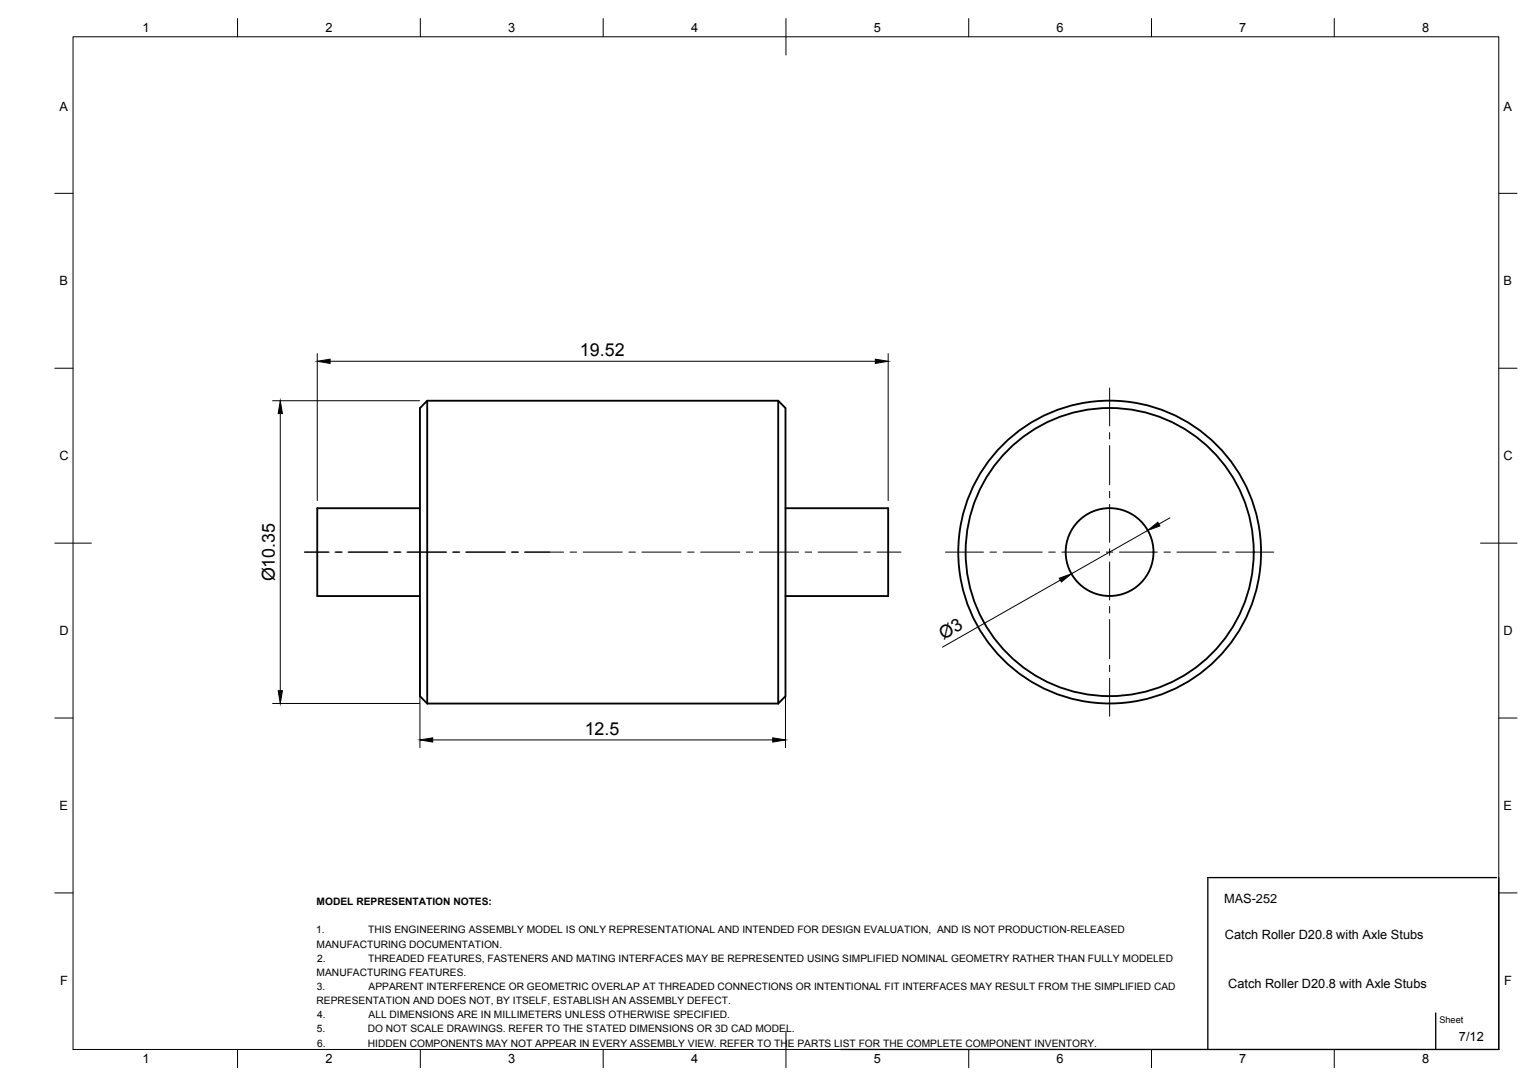
ISO-10303-21;
HEADER;
FILE_DESCRIPTION((''),'2;1');
FILE_NAME('Catch Roller D20.8 with Axle Stubs.step','2026-10-06T07:01:46+05:00',(''),(''),'','','');
FILE_SCHEMA (('AUTOMOTIVE_DESIGN { 1 0 10303 214 3 1 1 }'));
ENDSEC;
DATA;
#10=MECHANICAL_DESIGN_GEOMETRIC_PRESENTATION_REPRESENTATION('',(#142),#11396);
#97=CONICAL_SURFACE('',#6232,5.05,0.785398163397455) ;
#98=CONICAL_SURFACE('',#6236,5.05,0.785398163397455) ;
#112=SHAPE_REPRESENTATION_RELATIONSHIP('SRR','None',#11459,#127) ;
#127=ADVANCED_BREP_SHAPE_REPRESENTATION('',(#157),#11385) ;
#142=STYLED_ITEM('',(#11543),#157) ;
#157=MANIFOLD_SOLID_BREP('Catch Roller D20.8 with Axle Stubs',#5573) ;
#363=FACE_BOUND('',#1122,.T.) ;
#364=FACE_BOUND('',#1127,.T.) ;
#462=PLANE('',#6226) ;
#463=PLANE('',#6230) ;
#464=PLANE('',#6238) ;
#465=PLANE('',#6242) ;
#757=FACE_OUTER_BOUND('',#1119,.T.) ;
#758=FACE_OUTER_BOUND('',#1120,.T.) ;
#759=FACE_OUTER_BOUND('',#1121,.T.) ;
#760=FACE_OUTER_BOUND('',#1123,.T.) ;
#761=FACE_OUTER_BOUND('',#1124,.T.) ;
#762=FACE_OUTER_BOUND('',#1125,.T.) ;
#763=FACE_OUTER_BOUND('',#1126,.T.) ;
#764=FACE_OUTER_BOUND('',#1128,.T.) ;
#765=FACE_OUTER_BOUND('',#1129,.T.) ;
#1119=EDGE_LOOP('',(#4726)) ;
#1120=EDGE_LOOP('',(#4727,#4728,#4729,#4730)) ;
#1121=EDGE_LOOP('',(#4731)) ;
#1122=EDGE_LOOP('',(#4732)) ;
#1123=EDGE_LOOP('',(#4733,#4734,#4735,#4736)) ;
#1124=EDGE_LOOP('',(#4737,#4738,#4739,#4740)) ;
#1125=EDGE_LOOP('',(#4741,#4742,#4743,#4744)) ;
#1126=EDGE_LOOP('',(#4745)) ;
#1127=EDGE_LOOP('',(#4746)) ;
#1128=EDGE_LOOP('',(#4747,#4748,#4749,#4750)) ;
#1129=EDGE_LOOP('',(#4751)) ;
#1498=LINE('',#10819,#1881) ;
#1499=LINE('',#10826,#1882) ;
#1500=LINE('',#10830,#1883) ;
#1501=LINE('',#10834,#1884) ;
#1502=LINE('',#10841,#1885) ;
#1881=VECTOR('',#7652,1.5) ;
#1882=VECTOR('',#7661,5.05) ;
#1883=VECTOR('',#7666,5.175) ;
#1884=VECTOR('',#7671,5.05) ;
#1885=VECTOR('',#7680,1.5) ;
#2198=CIRCLE('',#6227,1.5) ;
#2199=CIRCLE('',#6229,1.5) ;
#2200=CIRCLE('',#6231,4.925) ;
#2201=CIRCLE('',#6233,5.175) ;
#2202=CIRCLE('',#6235,5.175) ;
#2203=CIRCLE('',#6237,4.925) ;
#2204=CIRCLE('',#6239,1.5) ;
#2205=CIRCLE('',#6241,1.5) ;
#2627=VERTEX_POINT('',#10814) ;
#2628=VERTEX_POINT('',#10817) ;
#2629=VERTEX_POINT('',#10821) ;
#2630=VERTEX_POINT('',#10824) ;
#2631=VERTEX_POINT('',#10828) ;
#2632=VERTEX_POINT('',#10832) ;
#2633=VERTEX_POINT('',#10836) ;
#2634=VERTEX_POINT('',#10839) ;
#3345=EDGE_CURVE('',#2627,#2627,#2198,.T.) ;
#3346=EDGE_CURVE('',#2628,#2628,#2199,.T.) ;
#3347=EDGE_CURVE('',#2628,#2627,#1498,.T.) ;
#3348=EDGE_CURVE('',#2629,#2629,#2200,.T.) ;
#3349=EDGE_CURVE('',#2630,#2630,#2201,.T.) ;
#3350=EDGE_CURVE('',#2630,#2629,#1499,.T.) ;
#3351=EDGE_CURVE('',#2631,#2631,#2202,.T.) ;
#3352=EDGE_CURVE('',#2631,#2630,#1500,.T.) ;
#3353=EDGE_CURVE('',#2632,#2632,#2203,.T.) ;
#3354=EDGE_CURVE('',#2632,#2631,#1501,.T.) ;
#3355=EDGE_CURVE('',#2633,#2633,#2204,.T.) ;
#3356=EDGE_CURVE('',#2634,#2634,#2205,.T.) ;
#3357=EDGE_CURVE('',#2634,#2633,#1502,.T.) ;
#4726=ORIENTED_EDGE('',*,*,#3345,.F.) ;
#4727=ORIENTED_EDGE('',*,*,#3346,.F.) ;
#4728=ORIENTED_EDGE('',*,*,#3347,.T.) ;
#4729=ORIENTED_EDGE('',*,*,#3345,.T.) ;
#4730=ORIENTED_EDGE('',*,*,#3347,.F.) ;
#4731=ORIENTED_EDGE('',*,*,#3348,.F.) ;
#4732=ORIENTED_EDGE('',*,*,#3346,.T.) ;
#4733=ORIENTED_EDGE('',*,*,#3349,.F.) ;
#4734=ORIENTED_EDGE('',*,*,#3350,.T.) ;
#4735=ORIENTED_EDGE('',*,*,#3348,.T.) ;
#4736=ORIENTED_EDGE('',*,*,#3350,.F.) ;
#4737=ORIENTED_EDGE('',*,*,#3351,.F.) ;
#4738=ORIENTED_EDGE('',*,*,#3352,.T.) ;
#4739=ORIENTED_EDGE('',*,*,#3349,.T.) ;
#4740=ORIENTED_EDGE('',*,*,#3352,.F.) ;
#4741=ORIENTED_EDGE('',*,*,#3353,.F.) ;
#4742=ORIENTED_EDGE('',*,*,#3354,.T.) ;
#4743=ORIENTED_EDGE('',*,*,#3351,.T.) ;
#4744=ORIENTED_EDGE('',*,*,#3354,.F.) ;
#4745=ORIENTED_EDGE('',*,*,#3353,.T.) ;
#4746=ORIENTED_EDGE('',*,*,#3355,.F.) ;
#4747=ORIENTED_EDGE('',*,*,#3356,.F.) ;
#4748=ORIENTED_EDGE('',*,*,#3357,.T.) ;
#4749=ORIENTED_EDGE('',*,*,#3355,.T.) ;
#4750=ORIENTED_EDGE('',*,*,#3357,.F.) ;
#4751=ORIENTED_EDGE('',*,*,#3356,.T.) ;
#5205=CYLINDRICAL_SURFACE('',#6228,1.5) ;
#5206=CYLINDRICAL_SURFACE('',#6234,5.175) ;
#5207=CYLINDRICAL_SURFACE('',#6240,1.5) ;
#5482=ADVANCED_FACE('',(#757),#462,.T.) ;
#5483=ADVANCED_FACE('',(#758),#5205,.T.) ;
#5484=ADVANCED_FACE('',(#759,#363),#463,.T.) ;
#5485=ADVANCED_FACE('',(#760),#97,.T.) ;
#5486=ADVANCED_FACE('',(#761),#5206,.T.) ;
#5487=ADVANCED_FACE('',(#762),#98,.T.) ;
#5488=ADVANCED_FACE('',(#763,#364),#464,.T.) ;
#5489=ADVANCED_FACE('',(#764),#5207,.T.) ;
#5490=ADVANCED_FACE('',(#765),#465,.T.) ;
#5573=CLOSED_SHELL('',(#5482,#5483,#5484,#5485,#5486,#5487,#5488,#5489,
#5490)) ;
#6225=AXIS2_PLACEMENT_3D('',#10812,#7642,#7643) ;
#6226=AXIS2_PLACEMENT_3D('',#10813,#7644,#7645) ;
#6227=AXIS2_PLACEMENT_3D('',#10815,#7646,#7647) ;
#6228=AXIS2_PLACEMENT_3D('',#10816,#7648,#7649) ;
#6229=AXIS2_PLACEMENT_3D('',#10818,#7650,#7651) ;
#6230=AXIS2_PLACEMENT_3D('',#10820,#7653,#7654) ;
#6231=AXIS2_PLACEMENT_3D('',#10822,#7655,#7656) ;
#6232=AXIS2_PLACEMENT_3D('',#10823,#7657,#7658) ;
#6233=AXIS2_PLACEMENT_3D('',#10825,#7659,#7660) ;
#6234=AXIS2_PLACEMENT_3D('',#10827,#7662,#7663) ;
#6235=AXIS2_PLACEMENT_3D('',#10829,#7664,#7665) ;
#6236=AXIS2_PLACEMENT_3D('',#10831,#7667,#7668) ;
#6237=AXIS2_PLACEMENT_3D('',#10833,#7669,#7670) ;
#6238=AXIS2_PLACEMENT_3D('',#10835,#7672,#7673) ;
#6239=AXIS2_PLACEMENT_3D('',#10837,#7674,#7675) ;
#6240=AXIS2_PLACEMENT_3D('',#10838,#7676,#7677) ;
#6241=AXIS2_PLACEMENT_3D('',#10840,#7678,#7679) ;
#6242=AXIS2_PLACEMENT_3D('',#10842,#7681,#7682) ;
#7642=DIRECTION('axis',(0.,0.,1.)) ;
#7643=DIRECTION('refdir',(1.,0.,0.)) ;
#7644=DIRECTION('center_axis',(-1.,0.,0.)) ;
#7645=DIRECTION('ref_axis',(0.,0.,1.)) ;
#7646=DIRECTION('center_axis',(1.,0.,0.)) ;
#7647=DIRECTION('ref_axis',(0.,0.,-1.)) ;
#7648=DIRECTION('center_axis',(1.,0.,0.)) ;
#7649=DIRECTION('ref_axis',(0.,1.,0.)) ;
#7650=DIRECTION('center_axis',(1.,0.,0.)) ;
#7651=DIRECTION('ref_axis',(0.,0.,-1.)) ;
#7652=DIRECTION('',(-1.,0.,0.)) ;
#7653=DIRECTION('center_axis',(-1.,0.,0.)) ;
#7654=DIRECTION('ref_axis',(0.,0.,1.)) ;
#7655=DIRECTION('center_axis',(1.,0.,0.)) ;
#7656=DIRECTION('ref_axis',(0.,0.,-1.)) ;
#7657=DIRECTION('center_axis',(1.,0.,0.)) ;
#7658=DIRECTION('ref_axis',(0.,1.,0.)) ;
#7659=DIRECTION('center_axis',(1.,0.,0.)) ;
#7660=DIRECTION('ref_axis',(0.,0.,-1.)) ;
#7661=DIRECTION('',(-0.707106781186543,0.707106781186552,8.65956056235499E-17)) ;
#7662=DIRECTION('center_axis',(1.,0.,0.)) ;
#7663=DIRECTION('ref_axis',(0.,1.,0.)) ;
#7664=DIRECTION('center_axis',(1.,0.,0.)) ;
#7665=DIRECTION('ref_axis',(0.,0.,-1.)) ;
#7666=DIRECTION('',(-1.,0.,0.)) ;
#7667=DIRECTION('center_axis',(-1.,0.,0.)) ;
#7668=DIRECTION('ref_axis',(0.,1.,0.)) ;
#7669=DIRECTION('center_axis',(1.,0.,0.)) ;
#7670=DIRECTION('ref_axis',(0.,0.,-1.)) ;
#7671=DIRECTION('',(-0.707106781186543,-0.707106781186552,-8.65956056235499E-17)) ;
#7672=DIRECTION('center_axis',(1.,0.,0.)) ;
#7673=DIRECTION('ref_axis',(0.,0.,-1.)) ;
#7674=DIRECTION('center_axis',(1.,0.,0.)) ;
#7675=DIRECTION('ref_axis',(0.,0.,-1.)) ;
#7676=DIRECTION('center_axis',(1.,0.,0.)) ;
#7677=DIRECTION('ref_axis',(0.,1.,0.)) ;
#7678=DIRECTION('center_axis',(1.,0.,0.)) ;
#7679=DIRECTION('ref_axis',(0.,0.,-1.)) ;
#7680=DIRECTION('',(-1.,0.,0.)) ;
#7681=DIRECTION('center_axis',(1.,0.,0.)) ;
#7682=DIRECTION('ref_axis',(0.,0.,-1.)) ;
#10812=CARTESIAN_POINT('',(0.,0.,0.)) ;
#10813=CARTESIAN_POINT('Origin',(-9.76,21.29,38.695)) ;
#10814=CARTESIAN_POINT('',(-9.76,18.29,38.695)) ;
#10815=CARTESIAN_POINT('Origin',(-9.76,19.79,38.695)) ;
#10816=CARTESIAN_POINT('Origin',(-8.005,19.79,38.695)) ;
#10817=CARTESIAN_POINT('',(-6.25,18.29,38.695)) ;
#10818=CARTESIAN_POINT('Origin',(-6.25,19.79,38.695)) ;
#10819=CARTESIAN_POINT('',(-8.005,18.29,38.695)) ;
#10820=CARTESIAN_POINT('Origin',(-6.25,24.715,38.695)) ;
#10821=CARTESIAN_POINT('',(-6.25,14.865,38.695)) ;
#10822=CARTESIAN_POINT('Origin',(-6.25,19.79,38.695)) ;
#10823=CARTESIAN_POINT('Origin',(-6.125,19.79,38.695)) ;
#10824=CARTESIAN_POINT('',(-6.,14.615,38.695)) ;
#10825=CARTESIAN_POINT('Origin',(-6.,19.79,38.695)) ;
#10826=CARTESIAN_POINT('',(-6.125,14.74,38.695)) ;
#10827=CARTESIAN_POINT('Origin',(0.,19.79,38.695)) ;
#10828=CARTESIAN_POINT('',(6.,14.615,38.695)) ;
#10829=CARTESIAN_POINT('Origin',(6.,19.79,38.695)) ;
#10830=CARTESIAN_POINT('',(0.,14.615,38.695)) ;
#10831=CARTESIAN_POINT('Origin',(6.125,19.79,38.695)) ;
#10832=CARTESIAN_POINT('',(6.25,14.865,38.695)) ;
#10833=CARTESIAN_POINT('Origin',(6.25,19.79,38.695)) ;
#10834=CARTESIAN_POINT('',(6.125,14.74,38.695)) ;
#10835=CARTESIAN_POINT('Origin',(6.25,21.29,38.695)) ;
#10836=CARTESIAN_POINT('',(6.25,18.29,38.695)) ;
#10837=CARTESIAN_POINT('Origin',(6.25,19.79,38.695)) ;
#10838=CARTESIAN_POINT('Origin',(8.005,19.79,38.695)) ;
#10839=CARTESIAN_POINT('',(9.76,18.29,38.695)) ;
#10840=CARTESIAN_POINT('Origin',(9.76,19.79,38.695)) ;
#10841=CARTESIAN_POINT('',(8.005,18.29,38.695)) ;
#10842=CARTESIAN_POINT('Origin',(9.76,19.79,38.695)) ;
#11368=UNCERTAINTY_MEASURE_WITH_UNIT(LENGTH_MEASURE(0.01),#11397,
'DISTANCE_ACCURACY_VALUE',
'Maximum model space distance between geometric entities at asserted c
onnectivities') ;
#11379=UNCERTAINTY_MEASURE_WITH_UNIT(LENGTH_MEASURE(0.01),#11397,
'DISTANCE_ACCURACY_VALUE',
'Maximum model space distance between geometric entities at asserted c
onnectivities') ;
#11385=(
GEOMETRIC_REPRESENTATION_CONTEXT(3)
GLOBAL_UNCERTAINTY_ASSIGNED_CONTEXT((#11368))
GLOBAL_UNIT_ASSIGNED_CONTEXT((#11397,#11399,#11400))
REPRESENTATION_CONTEXT('','3D')
) ;
#11396=(
GEOMETRIC_REPRESENTATION_CONTEXT(3)
GLOBAL_UNCERTAINTY_ASSIGNED_CONTEXT((#11379))
GLOBAL_UNIT_ASSIGNED_CONTEXT((#11397,#11399,#11400))
REPRESENTATION_CONTEXT('','3D')
) ;
#11397=(
LENGTH_UNIT()
NAMED_UNIT(*)
SI_UNIT(.MILLI.,.METRE.)
) ;
#11399=(
NAMED_UNIT(*)
PLANE_ANGLE_UNIT()
SI_UNIT($,.RADIAN.)
) ;
#11400=(
NAMED_UNIT(*)
SI_UNIT($,.STERADIAN.)
SOLID_ANGLE_UNIT()
) ;
#11406=SHAPE_DEFINITION_REPRESENTATION(#11422,#11459) ;
#11422=PRODUCT_DEFINITION_SHAPE('',$,#11476) ;
#11459=SHAPE_REPRESENTATION('',(#6225),#11385) ;
#11470=PRODUCT_DEFINITION_CONTEXT('part definition',#11520,'design') ;
#11476=PRODUCT_DEFINITION('Catch Roller D20.8 with Axle Stubs',
'Catch Roller D20.8 with Axle Stubs',#11492,#11470) ;
#11492=PRODUCT_DEFINITION_FORMATION('',$,#11527) ;
#11520=APPLICATION_CONTEXT(
'Core Data for Automotive Mechanical Design Process') ;
#11521=PRODUCT_CONTEXT('part definition',#11520,'mechanical') ;
#11527=PRODUCT('Catch Roller D20.8 with Axle Stubs',
'Catch Roller D20.8 with Axle Stubs',$,(#11521)) ;
#11543=PRESENTATION_STYLE_ASSIGNMENT((#11559)) ;
#11559=SURFACE_STYLE_USAGE(.BOTH.,#11575) ;
#11575=SURFACE_SIDE_STYLE('',(#11591)) ;
#11591=SURFACE_STYLE_FILL_AREA(#11607) ;
#11607=FILL_AREA_STYLE(
'MAS-252 Metallic - Catch Roller D20.8 with Axle Stubs',(#11623)) ;
#11623=FILL_AREA_STYLE_COLOUR(
'MAS-252 Metallic - Catch Roller D20.8 with Axle Stubs',#11639) ;
#11639=COLOUR_RGB(
'MAS-252 Metallic - Catch Roller D20.8 with Axle Stubs', 0.72549020, 0.75294118, 0.79215686) ;
ENDSEC;
END-ISO-10303-21;
